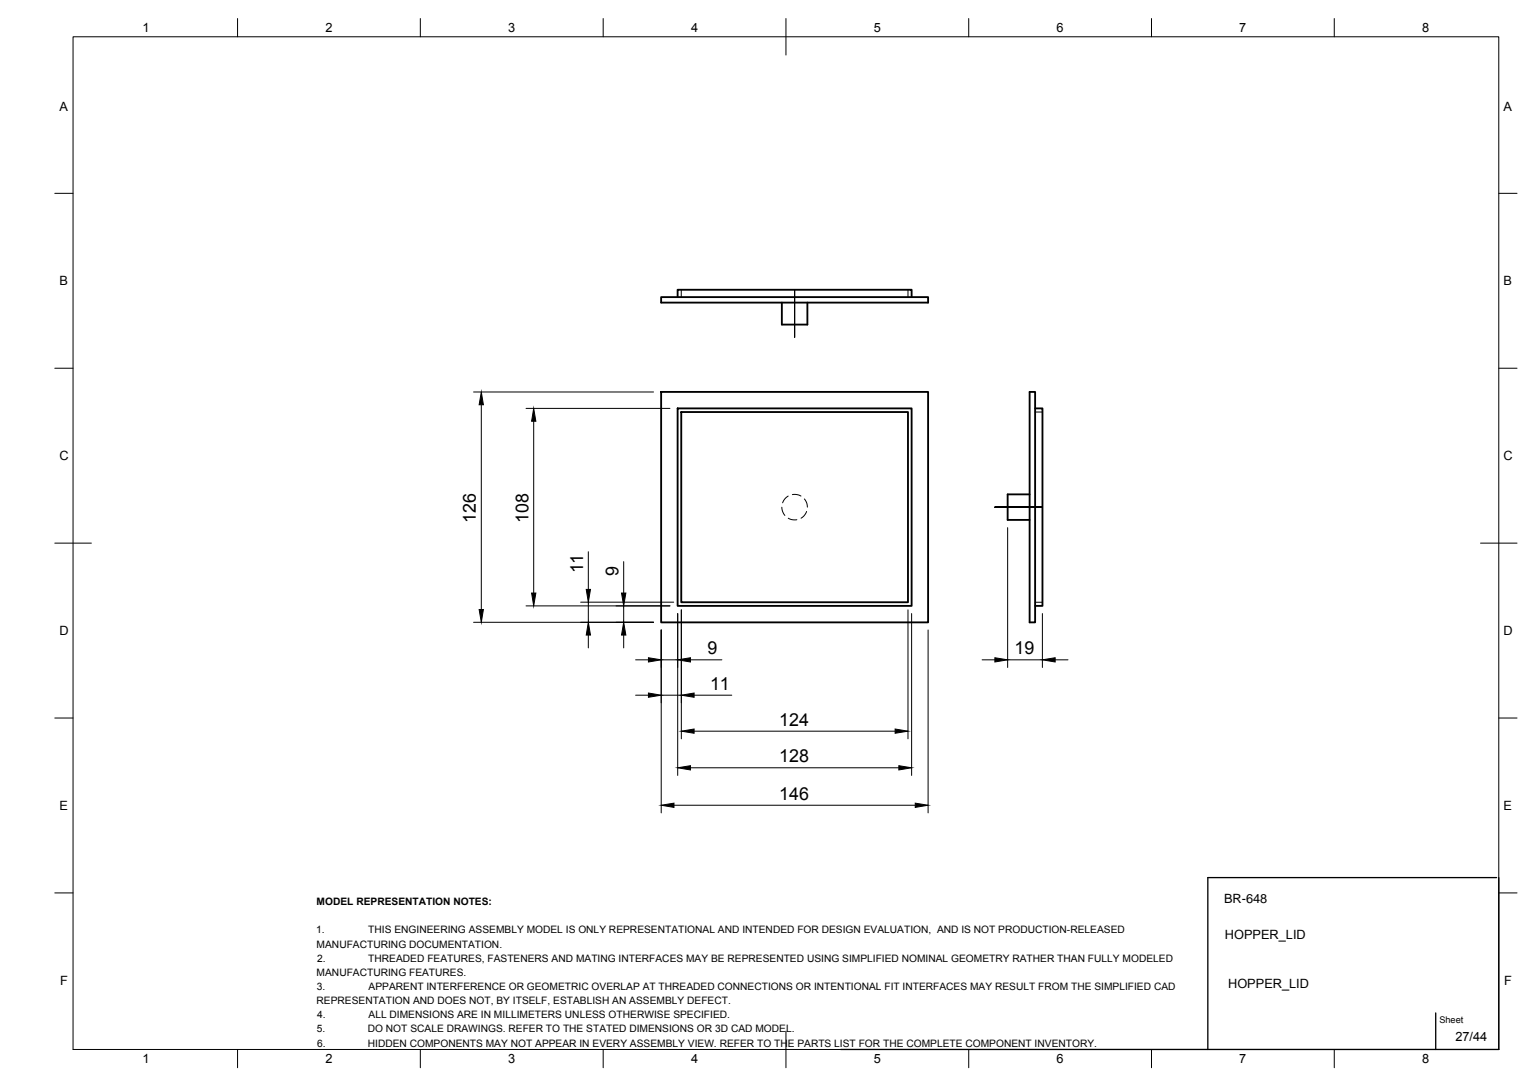
ISO-10303-21;
HEADER;
FILE_DESCRIPTION((''),'2;1');
FILE_NAME('HOPPER_LID.step','2026-10-01T22:05:39-07:00',(''),(''),'','','');
FILE_SCHEMA (('AUTOMOTIVE_DESIGN { 1 0 10303 214 3 1 1 }'));
ENDSEC;
DATA;
#10=MECHANICAL_DESIGN_GEOMETRIC_PRESENTATION_REPRESENTATION('',(#625),#24628);
#541=SHAPE_REPRESENTATION_RELATIONSHIP('SRR','None',#24814,#583) ;
#583=ADVANCED_BREP_SHAPE_REPRESENTATION('',(#664),#24604) ;
#625=STYLED_ITEM('',(#25038),#664) ;
#664=MANIFOLD_SOLID_BREP('HOPPER_LID',#13167) ;
#873=FACE_BOUND('',#4417,.T.) ;
#874=FACE_BOUND('',#4423,.T.) ;
#875=FACE_BOUND('',#4425,.T.) ;
#1450=LINE('',#22844,#2286) ;
#1451=LINE('',#22850,#2287) ;
#1452=LINE('',#22852,#2288) ;
#1453=LINE('',#22854,#2289) ;
#1454=LINE('',#22855,#2290) ;
#1455=LINE('',#22858,#2291) ;
#1456=LINE('',#22860,#2292) ;
#1457=LINE('',#22861,#2293) ;
#1458=LINE('',#22864,#2294) ;
#1459=LINE('',#22865,#2295) ;
#1460=LINE('',#22868,#2296) ;
#1461=LINE('',#22869,#2297) ;
#1462=LINE('',#22871,#2298) ;
#1463=LINE('',#22875,#2299) ;
#1464=LINE('',#22877,#2300) ;
#1465=LINE('',#22879,#2301) ;
#1466=LINE('',#22880,#2302) ;
#1467=LINE('',#22883,#2303) ;
#1468=LINE('',#22885,#2304) ;
#1469=LINE('',#22886,#2305) ;
#1470=LINE('',#22889,#2306) ;
#1471=LINE('',#22890,#2307) ;
#1472=LINE('',#22893,#2308) ;
#1473=LINE('',#22894,#2309) ;
#1474=LINE('',#22896,#2310) ;
#1475=LINE('',#22900,#2311) ;
#1476=LINE('',#22902,#2312) ;
#1477=LINE('',#22904,#2313) ;
#1478=LINE('',#22905,#2314) ;
#1479=LINE('',#22909,#2315) ;
#1480=LINE('',#22911,#2316) ;
#1481=LINE('',#22913,#2317) ;
#1482=LINE('',#22914,#2318) ;
#1483=LINE('',#22916,#2319) ;
#1484=LINE('',#22917,#2320) ;
#1485=LINE('',#22919,#2321) ;
#1486=LINE('',#22921,#2322) ;
#2286=VECTOR('',#18267,0.7) ;
#2287=VECTOR('',#18274,1.) ;
#2288=VECTOR('',#18275,1.) ;
#2289=VECTOR('',#18276,1.) ;
#2290=VECTOR('',#18277,1.) ;
#2291=VECTOR('',#18280,1.) ;
#2292=VECTOR('',#18281,1.) ;
#2293=VECTOR('',#18282,1.) ;
#2294=VECTOR('',#18285,1.) ;
#2295=VECTOR('',#18286,1.) ;
#2296=VECTOR('',#18289,1.) ;
#2297=VECTOR('',#18290,1.) ;
#2298=VECTOR('',#18293,1.) ;
#2299=VECTOR('',#18296,1.) ;
#2300=VECTOR('',#18297,1.) ;
#2301=VECTOR('',#18298,1.) ;
#2302=VECTOR('',#18299,1.) ;
#2303=VECTOR('',#18302,1.) ;
#2304=VECTOR('',#18303,1.) ;
#2305=VECTOR('',#18304,1.) ;
#2306=VECTOR('',#18307,1.) ;
#2307=VECTOR('',#18308,1.) ;
#2308=VECTOR('',#18311,1.) ;
#2309=VECTOR('',#18312,1.) ;
#2310=VECTOR('',#18315,1.) ;
#2311=VECTOR('',#18318,1.) ;
#2312=VECTOR('',#18319,1.) ;
#2313=VECTOR('',#18320,1.) ;
#2314=VECTOR('',#18321,1.) ;
#2315=VECTOR('',#18324,1.) ;
#2316=VECTOR('',#18325,1.) ;
#2317=VECTOR('',#18326,1.) ;
#2318=VECTOR('',#18327,1.) ;
#2319=VECTOR('',#18330,1.) ;
#2320=VECTOR('',#18331,1.) ;
#2321=VECTOR('',#18334,1.) ;
#2322=VECTOR('',#18337,1.) ;
#2874=CYLINDRICAL_SURFACE('',#14864,0.7) ;
#3455=FACE_OUTER_BOUND('',#4409,.T.) ;
#3456=FACE_OUTER_BOUND('',#4410,.T.) ;
#3457=FACE_OUTER_BOUND('',#4411,.T.) ;
#3458=FACE_OUTER_BOUND('',#4412,.T.) ;
#3459=FACE_OUTER_BOUND('',#4413,.T.) ;
#3460=FACE_OUTER_BOUND('',#4414,.T.) ;
#3461=FACE_OUTER_BOUND('',#4415,.T.) ;
#3462=FACE_OUTER_BOUND('',#4416,.T.) ;
#3463=FACE_OUTER_BOUND('',#4418,.T.) ;
#3464=FACE_OUTER_BOUND('',#4419,.T.) ;
#3465=FACE_OUTER_BOUND('',#4420,.T.) ;
#3466=FACE_OUTER_BOUND('',#4421,.T.) ;
#3467=FACE_OUTER_BOUND('',#4422,.T.) ;
#3468=FACE_OUTER_BOUND('',#4424,.T.) ;
#3469=FACE_OUTER_BOUND('',#4426,.T.) ;
#3470=FACE_OUTER_BOUND('',#4427,.T.) ;
#3471=FACE_OUTER_BOUND('',#4428,.T.) ;
#3472=FACE_OUTER_BOUND('',#4429,.T.) ;
#4409=EDGE_LOOP('',(#10785,#10786,#10787,#10788)) ;
#4410=EDGE_LOOP('',(#10789)) ;
#4411=EDGE_LOOP('',(#10790,#10791,#10792,#10793)) ;
#4412=EDGE_LOOP('',(#10794,#10795,#10796,#10797)) ;
#4413=EDGE_LOOP('',(#10798,#10799,#10800,#10801)) ;
#4414=EDGE_LOOP('',(#10802,#10803,#10804,#10805)) ;
#4415=EDGE_LOOP('',(#10806,#10807,#10808,#10809)) ;
#4416=EDGE_LOOP('',(#10810,#10811,#10812,#10813)) ;
#4417=EDGE_LOOP('',(#10814,#10815,#10816,#10817)) ;
#4418=EDGE_LOOP('',(#10818,#10819,#10820,#10821)) ;
#4419=EDGE_LOOP('',(#10822,#10823,#10824,#10825)) ;
#4420=EDGE_LOOP('',(#10826,#10827,#10828,#10829)) ;
#4421=EDGE_LOOP('',(#10830,#10831,#10832,#10833)) ;
#4422=EDGE_LOOP('',(#10834,#10835,#10836,#10837)) ;
#4423=EDGE_LOOP('',(#10838)) ;
#4424=EDGE_LOOP('',(#10839,#10840,#10841,#10842)) ;
#4425=EDGE_LOOP('',(#10843,#10844,#10845,#10846)) ;
#4426=EDGE_LOOP('',(#10847,#10848,#10849,#10850)) ;
#4427=EDGE_LOOP('',(#10851,#10852,#10853,#10854)) ;
#4428=EDGE_LOOP('',(#10855,#10856,#10857,#10858)) ;
#4429=EDGE_LOOP('',(#10859,#10860,#10861,#10862)) ;
#5346=CIRCLE('',#14865,0.7) ;
#5347=CIRCLE('',#14866,0.7) ;
#6332=VERTEX_POINT('',#22841) ;
#6333=VERTEX_POINT('',#22843) ;
#6334=VERTEX_POINT('',#22848) ;
#6335=VERTEX_POINT('',#22849) ;
#6336=VERTEX_POINT('',#22851) ;
#6337=VERTEX_POINT('',#22853) ;
#6338=VERTEX_POINT('',#22857) ;
#6339=VERTEX_POINT('',#22859) ;
#6340=VERTEX_POINT('',#22863) ;
#6341=VERTEX_POINT('',#22867) ;
#6342=VERTEX_POINT('',#22873) ;
#6343=VERTEX_POINT('',#22874) ;
#6344=VERTEX_POINT('',#22876) ;
#6345=VERTEX_POINT('',#22878) ;
#6346=VERTEX_POINT('',#22882) ;
#6347=VERTEX_POINT('',#22884) ;
#6348=VERTEX_POINT('',#22888) ;
#6349=VERTEX_POINT('',#22892) ;
#6350=VERTEX_POINT('',#22898) ;
#6351=VERTEX_POINT('',#22899) ;
#6352=VERTEX_POINT('',#22901) ;
#6353=VERTEX_POINT('',#22903) ;
#6354=VERTEX_POINT('',#22907) ;
#6355=VERTEX_POINT('',#22908) ;
#6356=VERTEX_POINT('',#22910) ;
#6357=VERTEX_POINT('',#22912) ;
#7882=EDGE_CURVE('',#6332,#6332,#5346,.T.) ;
#7883=EDGE_CURVE('',#6332,#6333,#1450,.T.) ;
#7884=EDGE_CURVE('',#6333,#6333,#5347,.T.) ;
#7885=EDGE_CURVE('',#6334,#6335,#1451,.T.) ;
#7886=EDGE_CURVE('',#6336,#6334,#1452,.T.) ;
#7887=EDGE_CURVE('',#6336,#6337,#1453,.T.) ;
#7888=EDGE_CURVE('',#6337,#6335,#1454,.T.) ;
#7889=EDGE_CURVE('',#6335,#6338,#1455,.T.) ;
#7890=EDGE_CURVE('',#6337,#6339,#1456,.T.) ;
#7891=EDGE_CURVE('',#6339,#6338,#1457,.T.) ;
#7892=EDGE_CURVE('',#6340,#6336,#1458,.T.) ;
#7893=EDGE_CURVE('',#6339,#6340,#1459,.T.) ;
#7894=EDGE_CURVE('',#6338,#6341,#1460,.T.) ;
#7895=EDGE_CURVE('',#6340,#6341,#1461,.T.) ;
#7896=EDGE_CURVE('',#6341,#6334,#1462,.T.) ;
#7897=EDGE_CURVE('',#6342,#6343,#1463,.T.) ;
#7898=EDGE_CURVE('',#6343,#6344,#1464,.T.) ;
#7899=EDGE_CURVE('',#6344,#6345,#1465,.T.) ;
#7900=EDGE_CURVE('',#6345,#6342,#1466,.T.) ;
#7901=EDGE_CURVE('',#6346,#6344,#1467,.T.) ;
#7902=EDGE_CURVE('',#6347,#6343,#1468,.T.) ;
#7903=EDGE_CURVE('',#6346,#6347,#1469,.T.) ;
#7904=EDGE_CURVE('',#6348,#6345,#1470,.T.) ;
#7905=EDGE_CURVE('',#6348,#6346,#1471,.T.) ;
#7906=EDGE_CURVE('',#6349,#6342,#1472,.T.) ;
#7907=EDGE_CURVE('',#6349,#6348,#1473,.T.) ;
#7908=EDGE_CURVE('',#6347,#6349,#1474,.T.) ;
#7909=EDGE_CURVE('',#6350,#6351,#1475,.T.) ;
#7910=EDGE_CURVE('',#6351,#6352,#1476,.T.) ;
#7911=EDGE_CURVE('',#6352,#6353,#1477,.T.) ;
#7912=EDGE_CURVE('',#6353,#6350,#1478,.T.) ;
#7913=EDGE_CURVE('',#6354,#6355,#1479,.T.) ;
#7914=EDGE_CURVE('',#6355,#6356,#1480,.T.) ;
#7915=EDGE_CURVE('',#6356,#6357,#1481,.T.) ;
#7916=EDGE_CURVE('',#6357,#6354,#1482,.T.) ;
#7917=EDGE_CURVE('',#6353,#6356,#1483,.T.) ;
#7918=EDGE_CURVE('',#6350,#6355,#1484,.T.) ;
#7919=EDGE_CURVE('',#6352,#6357,#1485,.T.) ;
#7920=EDGE_CURVE('',#6351,#6354,#1486,.T.) ;
#10785=ORIENTED_EDGE('',*,*,#7882,.F.) ;
#10786=ORIENTED_EDGE('',*,*,#7883,.T.) ;
#10787=ORIENTED_EDGE('',*,*,#7884,.F.) ;
#10788=ORIENTED_EDGE('',*,*,#7883,.F.) ;
#10789=ORIENTED_EDGE('',*,*,#7882,.T.) ;
#10790=ORIENTED_EDGE('',*,*,#7885,.F.) ;
#10791=ORIENTED_EDGE('',*,*,#7886,.F.) ;
#10792=ORIENTED_EDGE('',*,*,#7887,.T.) ;
#10793=ORIENTED_EDGE('',*,*,#7888,.T.) ;
#10794=ORIENTED_EDGE('',*,*,#7889,.F.) ;
#10795=ORIENTED_EDGE('',*,*,#7888,.F.) ;
#10796=ORIENTED_EDGE('',*,*,#7890,.T.) ;
#10797=ORIENTED_EDGE('',*,*,#7891,.T.) ;
#10798=ORIENTED_EDGE('',*,*,#7892,.F.) ;
#10799=ORIENTED_EDGE('',*,*,#7893,.F.) ;
#10800=ORIENTED_EDGE('',*,*,#7890,.F.) ;
#10801=ORIENTED_EDGE('',*,*,#7887,.F.) ;
#10802=ORIENTED_EDGE('',*,*,#7894,.F.) ;
#10803=ORIENTED_EDGE('',*,*,#7891,.F.) ;
#10804=ORIENTED_EDGE('',*,*,#7893,.T.) ;
#10805=ORIENTED_EDGE('',*,*,#7895,.T.) ;
#10806=ORIENTED_EDGE('',*,*,#7896,.F.) ;
#10807=ORIENTED_EDGE('',*,*,#7895,.F.) ;
#10808=ORIENTED_EDGE('',*,*,#7892,.T.) ;
#10809=ORIENTED_EDGE('',*,*,#7886,.T.) ;
#10810=ORIENTED_EDGE('',*,*,#7897,.T.) ;
#10811=ORIENTED_EDGE('',*,*,#7898,.T.) ;
#10812=ORIENTED_EDGE('',*,*,#7899,.T.) ;
#10813=ORIENTED_EDGE('',*,*,#7900,.T.) ;
#10814=ORIENTED_EDGE('',*,*,#7894,.T.) ;
#10815=ORIENTED_EDGE('',*,*,#7896,.T.) ;
#10816=ORIENTED_EDGE('',*,*,#7885,.T.) ;
#10817=ORIENTED_EDGE('',*,*,#7889,.T.) ;
#10818=ORIENTED_EDGE('',*,*,#7901,.T.) ;
#10819=ORIENTED_EDGE('',*,*,#7898,.F.) ;
#10820=ORIENTED_EDGE('',*,*,#7902,.F.) ;
#10821=ORIENTED_EDGE('',*,*,#7903,.F.) ;
#10822=ORIENTED_EDGE('',*,*,#7904,.T.) ;
#10823=ORIENTED_EDGE('',*,*,#7899,.F.) ;
#10824=ORIENTED_EDGE('',*,*,#7901,.F.) ;
#10825=ORIENTED_EDGE('',*,*,#7905,.F.) ;
#10826=ORIENTED_EDGE('',*,*,#7906,.T.) ;
#10827=ORIENTED_EDGE('',*,*,#7900,.F.) ;
#10828=ORIENTED_EDGE('',*,*,#7904,.F.) ;
#10829=ORIENTED_EDGE('',*,*,#7907,.F.) ;
#10830=ORIENTED_EDGE('',*,*,#7902,.T.) ;
#10831=ORIENTED_EDGE('',*,*,#7897,.F.) ;
#10832=ORIENTED_EDGE('',*,*,#7906,.F.) ;
#10833=ORIENTED_EDGE('',*,*,#7908,.F.) ;
#10834=ORIENTED_EDGE('',*,*,#7909,.T.) ;
#10835=ORIENTED_EDGE('',*,*,#7910,.T.) ;
#10836=ORIENTED_EDGE('',*,*,#7911,.T.) ;
#10837=ORIENTED_EDGE('',*,*,#7912,.T.) ;
#10838=ORIENTED_EDGE('',*,*,#7884,.T.) ;
#10839=ORIENTED_EDGE('',*,*,#7913,.T.) ;
#10840=ORIENTED_EDGE('',*,*,#7914,.T.) ;
#10841=ORIENTED_EDGE('',*,*,#7915,.T.) ;
#10842=ORIENTED_EDGE('',*,*,#7916,.T.) ;
#10843=ORIENTED_EDGE('',*,*,#7903,.T.) ;
#10844=ORIENTED_EDGE('',*,*,#7908,.T.) ;
#10845=ORIENTED_EDGE('',*,*,#7907,.T.) ;
#10846=ORIENTED_EDGE('',*,*,#7905,.T.) ;
#10847=ORIENTED_EDGE('',*,*,#7917,.T.) ;
#10848=ORIENTED_EDGE('',*,*,#7914,.F.) ;
#10849=ORIENTED_EDGE('',*,*,#7918,.F.) ;
#10850=ORIENTED_EDGE('',*,*,#7912,.F.) ;
#10851=ORIENTED_EDGE('',*,*,#7919,.T.) ;
#10852=ORIENTED_EDGE('',*,*,#7915,.F.) ;
#10853=ORIENTED_EDGE('',*,*,#7917,.F.) ;
#10854=ORIENTED_EDGE('',*,*,#7911,.F.) ;
#10855=ORIENTED_EDGE('',*,*,#7920,.T.) ;
#10856=ORIENTED_EDGE('',*,*,#7916,.F.) ;
#10857=ORIENTED_EDGE('',*,*,#7919,.F.) ;
#10858=ORIENTED_EDGE('',*,*,#7910,.F.) ;
#10859=ORIENTED_EDGE('',*,*,#7918,.T.) ;
#10860=ORIENTED_EDGE('',*,*,#7913,.F.) ;
#10861=ORIENTED_EDGE('',*,*,#7920,.F.) ;
#10862=ORIENTED_EDGE('',*,*,#7909,.F.) ;
#12166=PLANE('',#14867) ;
#12167=PLANE('',#14868) ;
#12168=PLANE('',#14869) ;
#12169=PLANE('',#14870) ;
#12170=PLANE('',#14871) ;
#12171=PLANE('',#14872) ;
#12172=PLANE('',#14873) ;
#12173=PLANE('',#14874) ;
#12174=PLANE('',#14875) ;
#12175=PLANE('',#14876) ;
#12176=PLANE('',#14877) ;
#12177=PLANE('',#14878) ;
#12178=PLANE('',#14879) ;
#12179=PLANE('',#14880) ;
#12180=PLANE('',#14881) ;
#12181=PLANE('',#14882) ;
#12182=PLANE('',#14883) ;
#12850=ADVANCED_FACE('',(#3455),#2874,.T.) ;
#12851=ADVANCED_FACE('',(#3456),#12166,.T.) ;
#12852=ADVANCED_FACE('',(#3457),#12167,.T.) ;
#12853=ADVANCED_FACE('',(#3458),#12168,.T.) ;
#12854=ADVANCED_FACE('',(#3459),#12169,.F.) ;
#12855=ADVANCED_FACE('',(#3460),#12170,.T.) ;
#12856=ADVANCED_FACE('',(#3461),#12171,.T.) ;
#12857=ADVANCED_FACE('',(#3462,#873),#12172,.F.) ;
#12858=ADVANCED_FACE('',(#3463),#12173,.F.) ;
#12859=ADVANCED_FACE('',(#3464),#12174,.F.) ;
#12860=ADVANCED_FACE('',(#3465),#12175,.F.) ;
#12861=ADVANCED_FACE('',(#3466),#12176,.F.) ;
#12862=ADVANCED_FACE('',(#3467,#874),#12177,.T.) ;
#12863=ADVANCED_FACE('',(#3468,#875),#12178,.F.) ;
#12864=ADVANCED_FACE('',(#3469),#12179,.F.) ;
#12865=ADVANCED_FACE('',(#3470),#12180,.F.) ;
#12866=ADVANCED_FACE('',(#3471),#12181,.F.) ;
#12867=ADVANCED_FACE('',(#3472),#12182,.F.) ;
#13167=CLOSED_SHELL('',(#12850,#12851,#12852,#12853,#12854,#12855,#12856,
#12857,#12858,#12859,#12860,#12861,#12862,#12863,#12864,#12865,#12866,#12867)) ;
#14863=AXIS2_PLACEMENT_3D('',#22839,#18261,#18262) ;
#14864=AXIS2_PLACEMENT_3D('',#22840,#18263,#18264) ;
#14865=AXIS2_PLACEMENT_3D('',#22842,#18265,#18266) ;
#14866=AXIS2_PLACEMENT_3D('',#22845,#18268,#18269) ;
#14867=AXIS2_PLACEMENT_3D('',#22846,#18270,#18271) ;
#14868=AXIS2_PLACEMENT_3D('',#22847,#18272,#18273) ;
#14869=AXIS2_PLACEMENT_3D('',#22856,#18278,#18279) ;
#14870=AXIS2_PLACEMENT_3D('',#22862,#18283,#18284) ;
#14871=AXIS2_PLACEMENT_3D('',#22866,#18287,#18288) ;
#14872=AXIS2_PLACEMENT_3D('',#22870,#18291,#18292) ;
#14873=AXIS2_PLACEMENT_3D('',#22872,#18294,#18295) ;
#14874=AXIS2_PLACEMENT_3D('',#22881,#18300,#18301) ;
#14875=AXIS2_PLACEMENT_3D('',#22887,#18305,#18306) ;
#14876=AXIS2_PLACEMENT_3D('',#22891,#18309,#18310) ;
#14877=AXIS2_PLACEMENT_3D('',#22895,#18313,#18314) ;
#14878=AXIS2_PLACEMENT_3D('',#22897,#18316,#18317) ;
#14879=AXIS2_PLACEMENT_3D('',#22906,#18322,#18323) ;
#14880=AXIS2_PLACEMENT_3D('',#22915,#18328,#18329) ;
#14881=AXIS2_PLACEMENT_3D('',#22918,#18332,#18333) ;
#14882=AXIS2_PLACEMENT_3D('',#22920,#18335,#18336) ;
#14883=AXIS2_PLACEMENT_3D('',#22922,#18338,#18339) ;
#18261=DIRECTION('axis',(0.,0.,1.)) ;
#18262=DIRECTION('refdir',(1.,0.,0.)) ;
#18263=DIRECTION('center_axis',(0.,0.,1.)) ;
#18264=DIRECTION('ref_axis',(1.,0.,0.)) ;
#18265=DIRECTION('center_axis',(0.,0.,1.)) ;
#18266=DIRECTION('ref_axis',(1.,0.,0.)) ;
#18267=DIRECTION('',(0.,0.,-1.)) ;
#18268=DIRECTION('center_axis',(0.,0.,-1.)) ;
#18269=DIRECTION('ref_axis',(1.,0.,0.)) ;
#18270=DIRECTION('center_axis',(0.,0.,1.)) ;
#18271=DIRECTION('ref_axis',(1.,0.,0.)) ;
#18272=DIRECTION('center_axis',(0.,-1.,0.)) ;
#18273=DIRECTION('ref_axis',(0.,0.,-1.)) ;
#18274=DIRECTION('',(-1.,0.,0.)) ;
#18275=DIRECTION('',(0.,0.,-1.)) ;
#18276=DIRECTION('',(-1.,0.,0.)) ;
#18277=DIRECTION('',(0.,0.,-1.)) ;
#18278=DIRECTION('center_axis',(1.,0.,0.)) ;
#18279=DIRECTION('ref_axis',(0.,0.,-1.)) ;
#18280=DIRECTION('',(0.,-1.,0.)) ;
#18281=DIRECTION('',(0.,-1.,0.)) ;
#18282=DIRECTION('',(0.,0.,-1.)) ;
#18283=DIRECTION('center_axis',(0.,0.,1.)) ;
#18284=DIRECTION('ref_axis',(1.,0.,0.)) ;
#18285=DIRECTION('',(0.,1.,0.)) ;
#18286=DIRECTION('',(1.,0.,0.)) ;
#18287=DIRECTION('center_axis',(0.,1.,0.)) ;
#18288=DIRECTION('ref_axis',(0.,0.,1.)) ;
#18289=DIRECTION('',(1.,0.,0.)) ;
#18290=DIRECTION('',(0.,0.,-1.)) ;
#18291=DIRECTION('center_axis',(-1.,0.,0.)) ;
#18292=DIRECTION('ref_axis',(0.,0.,1.)) ;
#18293=DIRECTION('',(0.,1.,0.)) ;
#18294=DIRECTION('center_axis',(0.,0.,1.)) ;
#18295=DIRECTION('ref_axis',(1.,0.,0.)) ;
#18296=DIRECTION('',(0.,-1.,0.)) ;
#18297=DIRECTION('',(-1.,0.,0.)) ;
#18298=DIRECTION('',(0.,1.,0.)) ;
#18299=DIRECTION('',(1.,0.,0.)) ;
#18300=DIRECTION('center_axis',(0.,1.,0.)) ;
#18301=DIRECTION('ref_axis',(0.,0.,1.)) ;
#18302=DIRECTION('',(0.,0.,-1.)) ;
#18303=DIRECTION('',(0.,0.,-1.)) ;
#18304=DIRECTION('',(1.,0.,0.)) ;
#18305=DIRECTION('center_axis',(1.,0.,0.)) ;
#18306=DIRECTION('ref_axis',(0.,0.,-1.)) ;
#18307=DIRECTION('',(0.,0.,-1.)) ;
#18308=DIRECTION('',(0.,-1.,0.)) ;
#18309=DIRECTION('center_axis',(0.,-1.,0.)) ;
#18310=DIRECTION('ref_axis',(0.,0.,-1.)) ;
#18311=DIRECTION('',(0.,0.,-1.)) ;
#18312=DIRECTION('',(-1.,0.,0.)) ;
#18313=DIRECTION('center_axis',(-1.,0.,0.)) ;
#18314=DIRECTION('ref_axis',(0.,0.,1.)) ;
#18315=DIRECTION('',(0.,1.,0.)) ;
#18316=DIRECTION('center_axis',(0.,0.,1.)) ;
#18317=DIRECTION('ref_axis',(1.,0.,0.)) ;
#18318=DIRECTION('',(0.,1.,0.)) ;
#18319=DIRECTION('',(-1.,0.,0.)) ;
#18320=DIRECTION('',(0.,-1.,0.)) ;
#18321=DIRECTION('',(1.,0.,0.)) ;
#18322=DIRECTION('center_axis',(0.,0.,1.)) ;
#18323=DIRECTION('ref_axis',(1.,0.,0.)) ;
#18324=DIRECTION('',(0.,-1.,0.)) ;
#18325=DIRECTION('',(-1.,0.,0.)) ;
#18326=DIRECTION('',(0.,1.,0.)) ;
#18327=DIRECTION('',(1.,0.,0.)) ;
#18328=DIRECTION('center_axis',(0.,1.,0.)) ;
#18329=DIRECTION('ref_axis',(0.,0.,1.)) ;
#18330=DIRECTION('',(0.,0.,-1.)) ;
#18331=DIRECTION('',(0.,0.,-1.)) ;
#18332=DIRECTION('center_axis',(1.,0.,0.)) ;
#18333=DIRECTION('ref_axis',(0.,0.,-1.)) ;
#18334=DIRECTION('',(0.,0.,-1.)) ;
#18335=DIRECTION('center_axis',(0.,-1.,0.)) ;
#18336=DIRECTION('ref_axis',(0.,0.,-1.)) ;
#18337=DIRECTION('',(0.,0.,-1.)) ;
#18338=DIRECTION('center_axis',(-1.,0.,0.)) ;
#18339=DIRECTION('ref_axis',(0.,0.,1.)) ;
#22839=CARTESIAN_POINT('',(0.,0.,0.)) ;
#22840=CARTESIAN_POINT('Origin',(-23.,-1.8,15.9)) ;
#22841=CARTESIAN_POINT('',(-23.7,-1.8,16.5)) ;
#22842=CARTESIAN_POINT('Origin',(-23.,-1.8,16.5)) ;
#22843=CARTESIAN_POINT('',(-23.7,-1.8,15.3)) ;
#22844=CARTESIAN_POINT('',(-23.7,-1.8,15.9)) ;
#22845=CARTESIAN_POINT('Origin',(-23.,-1.8,15.3)) ;
#22846=CARTESIAN_POINT('Origin',(-23.,-1.8,16.5)) ;
#22847=CARTESIAN_POINT('Origin',(-23.,3.4,14.75)) ;
#22848=CARTESIAN_POINT('',(-16.8,3.4,14.6)) ;
#22849=CARTESIAN_POINT('',(-29.2,3.4,14.6)) ;
#22850=CARTESIAN_POINT('',(-23.,3.4,14.6)) ;
#22851=CARTESIAN_POINT('',(-16.8,3.4,15.)) ;
#22852=CARTESIAN_POINT('',(-16.8,3.4,14.75)) ;
#22853=CARTESIAN_POINT('',(-29.2,3.4,15.)) ;
#22854=CARTESIAN_POINT('',(-23.,3.4,15.)) ;
#22855=CARTESIAN_POINT('',(-29.2,3.4,14.75)) ;
#22856=CARTESIAN_POINT('Origin',(-29.2,-1.8,14.75)) ;
#22857=CARTESIAN_POINT('',(-29.2,-7.,14.6)) ;
#22858=CARTESIAN_POINT('',(-29.2,-1.8,14.6)) ;
#22859=CARTESIAN_POINT('',(-29.2,-7.,15.)) ;
#22860=CARTESIAN_POINT('',(-29.2,-1.8,15.)) ;
#22861=CARTESIAN_POINT('',(-29.2,-7.,14.75)) ;
#22862=CARTESIAN_POINT('Origin',(-23.,-1.8,15.)) ;
#22863=CARTESIAN_POINT('',(-16.8,-7.,15.)) ;
#22864=CARTESIAN_POINT('',(-16.8,-1.8,15.)) ;
#22865=CARTESIAN_POINT('',(-23.,-7.,15.)) ;
#22866=CARTESIAN_POINT('Origin',(-23.,-7.,14.75)) ;
#22867=CARTESIAN_POINT('',(-16.8,-7.,14.6)) ;
#22868=CARTESIAN_POINT('',(-23.,-7.,14.6)) ;
#22869=CARTESIAN_POINT('',(-16.8,-7.,14.75)) ;
#22870=CARTESIAN_POINT('Origin',(-16.8,-1.8,14.75)) ;
#22871=CARTESIAN_POINT('',(-16.8,-1.8,14.6)) ;
#22872=CARTESIAN_POINT('Origin',(-23.,-1.8,14.6)) ;
#22873=CARTESIAN_POINT('',(-16.6,3.6,14.6)) ;
#22874=CARTESIAN_POINT('',(-16.6,-7.2,14.6)) ;
#22875=CARTESIAN_POINT('',(-16.6,-1.8,14.6)) ;
#22876=CARTESIAN_POINT('',(-29.4,-7.2,14.6)) ;
#22877=CARTESIAN_POINT('',(-23.,-7.2,14.6)) ;
#22878=CARTESIAN_POINT('',(-29.4,3.6,14.6)) ;
#22879=CARTESIAN_POINT('',(-29.4,-1.8,14.6)) ;
#22880=CARTESIAN_POINT('',(-23.,3.6,14.6)) ;
#22881=CARTESIAN_POINT('Origin',(-23.,-7.2,14.8)) ;
#22882=CARTESIAN_POINT('',(-29.4,-7.2,15.)) ;
#22883=CARTESIAN_POINT('',(-29.4,-7.2,14.8)) ;
#22884=CARTESIAN_POINT('',(-16.6,-7.2,15.)) ;
#22885=CARTESIAN_POINT('',(-16.6,-7.2,14.8)) ;
#22886=CARTESIAN_POINT('',(-23.,-7.2,15.)) ;
#22887=CARTESIAN_POINT('Origin',(-29.4,-1.8,14.8)) ;
#22888=CARTESIAN_POINT('',(-29.4,3.6,15.)) ;
#22889=CARTESIAN_POINT('',(-29.4,3.6,14.8)) ;
#22890=CARTESIAN_POINT('',(-29.4,-1.8,15.)) ;
#22891=CARTESIAN_POINT('Origin',(-23.,3.6,14.8)) ;
#22892=CARTESIAN_POINT('',(-16.6,3.6,15.)) ;
#22893=CARTESIAN_POINT('',(-16.6,3.6,14.8)) ;
#22894=CARTESIAN_POINT('',(-23.,3.6,15.)) ;
#22895=CARTESIAN_POINT('Origin',(-16.6,-1.8,14.8)) ;
#22896=CARTESIAN_POINT('',(-16.6,-1.8,15.)) ;
#22897=CARTESIAN_POINT('Origin',(-23.,-1.8,15.3)) ;
#22898=CARTESIAN_POINT('',(-15.7,-8.1,15.3)) ;
#22899=CARTESIAN_POINT('',(-15.7,4.5,15.3)) ;
#22900=CARTESIAN_POINT('',(-15.7,-1.8,15.3)) ;
#22901=CARTESIAN_POINT('',(-30.3,4.5,15.3)) ;
#22902=CARTESIAN_POINT('',(-23.,4.5,15.3)) ;
#22903=CARTESIAN_POINT('',(-30.3,-8.1,15.3)) ;
#22904=CARTESIAN_POINT('',(-30.3,-1.8,15.3)) ;
#22905=CARTESIAN_POINT('',(-23.,-8.1,15.3)) ;
#22906=CARTESIAN_POINT('Origin',(-23.,-1.8,15.)) ;
#22907=CARTESIAN_POINT('',(-15.7,4.5,15.)) ;
#22908=CARTESIAN_POINT('',(-15.7,-8.1,15.)) ;
#22909=CARTESIAN_POINT('',(-15.7,-1.8,15.)) ;
#22910=CARTESIAN_POINT('',(-30.3,-8.1,15.)) ;
#22911=CARTESIAN_POINT('',(-23.,-8.1,15.)) ;
#22912=CARTESIAN_POINT('',(-30.3,4.5,15.)) ;
#22913=CARTESIAN_POINT('',(-30.3,-1.8,15.)) ;
#22914=CARTESIAN_POINT('',(-23.,4.5,15.)) ;
#22915=CARTESIAN_POINT('Origin',(-23.,-8.1,15.15)) ;
#22916=CARTESIAN_POINT('',(-30.3,-8.1,15.15)) ;
#22917=CARTESIAN_POINT('',(-15.7,-8.1,15.15)) ;
#22918=CARTESIAN_POINT('Origin',(-30.3,-1.8,15.15)) ;
#22919=CARTESIAN_POINT('',(-30.3,4.5,15.15)) ;
#22920=CARTESIAN_POINT('Origin',(-23.,4.5,15.15)) ;
#22921=CARTESIAN_POINT('',(-15.7,4.5,15.15)) ;
#22922=CARTESIAN_POINT('Origin',(-15.7,-1.8,15.15)) ;
#24556=UNCERTAINTY_MEASURE_WITH_UNIT(LENGTH_MEASURE(0.001),#24629,
'DISTANCE_ACCURACY_VALUE',
'Maximum model space distance between geometric entities at asserted c
onnectivities') ;
#24580=UNCERTAINTY_MEASURE_WITH_UNIT(LENGTH_MEASURE(0.001),#24629,
'DISTANCE_ACCURACY_VALUE',
'Maximum model space distance between geometric entities at asserted c
onnectivities') ;
#24604=(
GEOMETRIC_REPRESENTATION_CONTEXT(3)
GLOBAL_UNCERTAINTY_ASSIGNED_CONTEXT((#24556))
GLOBAL_UNIT_ASSIGNED_CONTEXT((#24629,#24631,#24632))
REPRESENTATION_CONTEXT('','3D')
) ;
#24628=(
GEOMETRIC_REPRESENTATION_CONTEXT(3)
GLOBAL_UNCERTAINTY_ASSIGNED_CONTEXT((#24580))
GLOBAL_UNIT_ASSIGNED_CONTEXT((#24629,#24631,#24632))
REPRESENTATION_CONTEXT('','3D')
) ;
#24629=(
LENGTH_UNIT()
NAMED_UNIT(*)
SI_UNIT(.CENTI.,.METRE.)
) ;
#24631=(
NAMED_UNIT(*)
PLANE_ANGLE_UNIT()
SI_UNIT($,.RADIAN.)
) ;
#24632=(
NAMED_UNIT(*)
SI_UNIT($,.STERADIAN.)
SOLID_ANGLE_UNIT()
) ;
#24656=SHAPE_DEFINITION_REPRESENTATION(#24725,#24814) ;
#24725=PRODUCT_DEFINITION_SHAPE('',$,#24862) ;
#24814=SHAPE_REPRESENTATION('',(#14863),#24604) ;
#24838=PRODUCT_DEFINITION_CONTEXT('part definition',#24981,'design') ;
#24862=PRODUCT_DEFINITION('HOPPER_LID','HOPPER_LID',#24909,
#24838) ;
#24909=PRODUCT_DEFINITION_FORMATION('',$,#25006) ;
#24981=APPLICATION_CONTEXT(
'Core Data for Automotive Mechanical Design Process') ;
#24982=PRODUCT_CONTEXT('part definition',#24981,'mechanical') ;
#25006=PRODUCT('HOPPER_LID','HOPPER_LID',$,(#24982)) ;
#25038=PRESENTATION_STYLE_ASSIGNMENT((#25048)) ;
#25048=SURFACE_STYLE_USAGE(.BOTH.,#25058) ;
#25058=SURFACE_SIDE_STYLE('',(#25068)) ;
#25068=SURFACE_STYLE_FILL_AREA(#25078) ;
#25078=FILL_AREA_STYLE('Surface - Matte',(#25088)) ;
#25088=FILL_AREA_STYLE_COLOUR('Surface - Matte',#25098) ;
#25098=COLOUR_RGB('Surface - Matte', 0.66274510, 0.83137255, 0.94901961) ;
ENDSEC;
END-ISO-10303-21;
